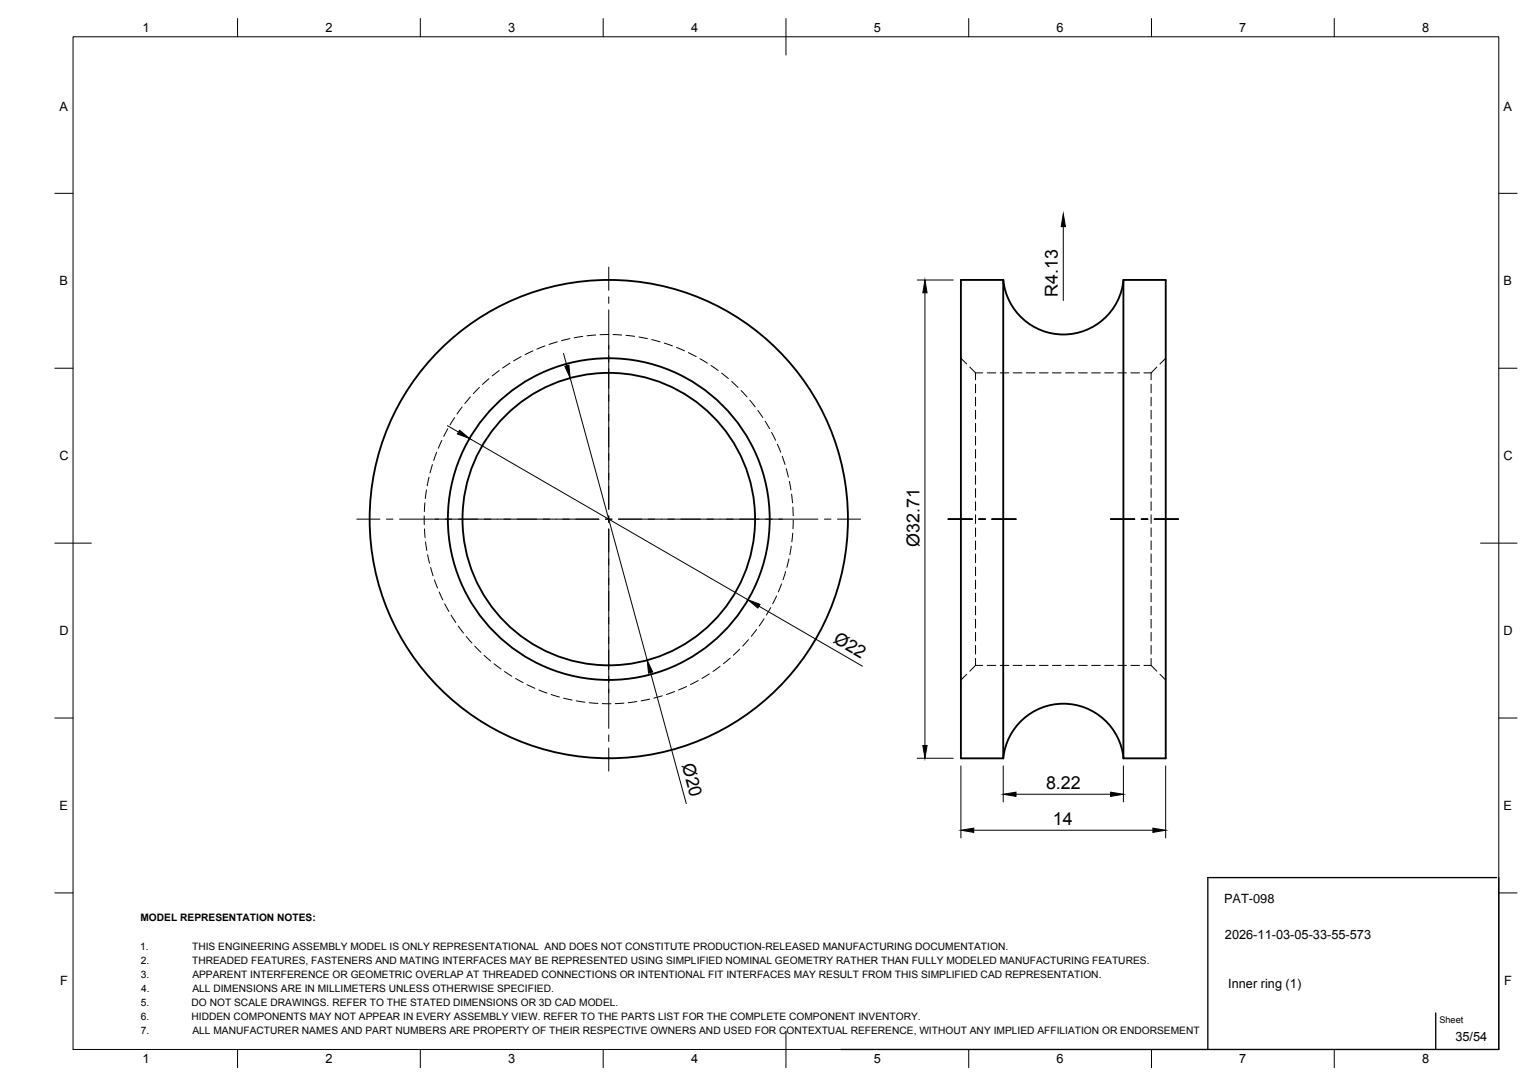
ISO-10303-21;
HEADER;
/* Generated by software containing ST-Developer
 * from STEP Tools, Inc. (www.steptools.com) 
 */

FILE_DESCRIPTION(
/* description */ ('Spring compression tester'),
/* implementation_level */ '2;1');

FILE_NAME(
/* name */ 'Inner ring (1).step',
/* time_stamp */ '2026-10-28T03:24:11-07:00',
/* author */ (''),
/* organization */ (''),
/* preprocessor_version */ 'ST-DEVELOPER v20.2',
/* originating_system */ 'Autodesk Translation Framework v15.17.0.0',
/* authorisation */ '');

FILE_SCHEMA (('AUTOMOTIVE_DESIGN { 1 0 10303 214 3 1 1 }'));
ENDSEC;

DATA;
#10=MECHANICAL_DESIGN_GEOMETRIC_PRESENTATION_REPRESENTATION('',(#1139),#43521);
#929=TOROIDAL_SURFACE('',#20122,1.675,0.412776);
#954=CONICAL_SURFACE('',#20133,1.05,0.785398163397449);
#955=CONICAL_SURFACE('',#20140,1.05,0.785398163397449);
#1012=SHAPE_REPRESENTATION_RELATIONSHIP('SRR','None',#43826,#1072);
#1072=ADVANCED_BREP_SHAPE_REPRESENTATION('',(#1213),#43486);
#1139=STYLED_ITEM('',(#44202),#1213);
#1213=MANIFOLD_SOLID_BREP('Body1',#18577);
#1459=FACE_BOUND('',#3908,.T.);
#1460=FACE_BOUND('',#3911,.T.);
#1904=PLANE('',#20135);
#1905=PLANE('',#20138);
#2644=FACE_OUTER_BOUND('',#3903,.T.);
#2645=FACE_OUTER_BOUND('',#3904,.T.);
#2646=FACE_OUTER_BOUND('',#3905,.T.);
#2647=FACE_OUTER_BOUND('',#3906,.T.);
#2648=FACE_OUTER_BOUND('',#3907,.T.);
#2649=FACE_OUTER_BOUND('',#3909,.T.);
#2650=FACE_OUTER_BOUND('',#3910,.T.);
#2651=FACE_OUTER_BOUND('',#3912,.T.);
#3903=EDGE_LOOP('',(#14319,#14320,#14321,#14322,#14323,#14324));
#3904=EDGE_LOOP('',(#14325,#14326,#14327,#14328,#14329));
#3905=EDGE_LOOP('',(#14330,#14331,#14332,#14333));
#3906=EDGE_LOOP('',(#14334,#14335,#14336,#14337));
#3907=EDGE_LOOP('',(#14338));
#3908=EDGE_LOOP('',(#14339));
#3909=EDGE_LOOP('',(#14340,#14341,#14342,#14343,#14344));
#3910=EDGE_LOOP('',(#14345));
#3911=EDGE_LOOP('',(#14346));
#3912=EDGE_LOOP('',(#14347,#14348,#14349,#14350));
#5317=LINE('',#29028,#6749);
#5318=LINE('',#29034,#6750);
#5319=LINE('',#29038,#6751);
#5320=LINE('',#29044,#6752);
#5321=LINE('',#29049,#6753);
#6749=VECTOR('',#23597,1.63531);
#6750=VECTOR('',#23604,1.);
#6751=VECTOR('',#23609,1.05);
#6752=VECTOR('',#23618,1.63531);
#6753=VECTOR('',#23625,1.05);
#7796=CIRCLE('',#20123,1.63531);
#7797=CIRCLE('',#20124,1.63531);
#7798=CIRCLE('',#20125,0.412776);
#7799=CIRCLE('',#20126,1.63531);
#7800=CIRCLE('',#20127,1.63531);
#7801=CIRCLE('',#20129,1.63531);
#7802=CIRCLE('',#20131,1.);
#7803=CIRCLE('',#20132,1.);
#7804=CIRCLE('',#20134,1.1);
#7805=CIRCLE('',#20137,1.63531);
#7806=CIRCLE('',#20139,1.1);
#8843=VERTEX_POINT('',#29017);
#8844=VERTEX_POINT('',#29018);
#8845=VERTEX_POINT('',#29021);
#8846=VERTEX_POINT('',#29023);
#8847=VERTEX_POINT('',#29027);
#8848=VERTEX_POINT('',#29031);
#8849=VERTEX_POINT('',#29033);
#8850=VERTEX_POINT('',#29037);
#8851=VERTEX_POINT('',#29042);
#8852=VERTEX_POINT('',#29046);
#10824=EDGE_CURVE('',#8843,#8844,#7796,.T.);
#10825=EDGE_CURVE('',#8844,#8843,#7797,.T.);
#10826=EDGE_CURVE('',#8844,#8845,#7798,.T.);
#10827=EDGE_CURVE('',#8846,#8845,#7799,.T.);
#10828=EDGE_CURVE('',#8845,#8846,#7800,.T.);
#10829=EDGE_CURVE('',#8846,#8847,#5317,.T.);
#10830=EDGE_CURVE('',#8847,#8847,#7801,.T.);
#10831=EDGE_CURVE('',#8848,#8848,#7802,.T.);
#10832=EDGE_CURVE('',#8848,#8849,#5318,.T.);
#10833=EDGE_CURVE('',#8849,#8849,#7803,.T.);
#10834=EDGE_CURVE('',#8849,#8850,#5319,.T.);
#10835=EDGE_CURVE('',#8850,#8850,#7804,.T.);
#10836=EDGE_CURVE('',#8851,#8851,#7805,.T.);
#10837=EDGE_CURVE('',#8851,#8843,#5320,.T.);
#10838=EDGE_CURVE('',#8852,#8852,#7806,.T.);
#10839=EDGE_CURVE('',#8852,#8848,#5321,.T.);
#14319=ORIENTED_EDGE('',*,*,#10824,.F.);
#14320=ORIENTED_EDGE('',*,*,#10825,.F.);
#14321=ORIENTED_EDGE('',*,*,#10826,.T.);
#14322=ORIENTED_EDGE('',*,*,#10827,.F.);
#14323=ORIENTED_EDGE('',*,*,#10828,.F.);
#14324=ORIENTED_EDGE('',*,*,#10826,.F.);
#14325=ORIENTED_EDGE('',*,*,#10827,.T.);
#14326=ORIENTED_EDGE('',*,*,#10828,.T.);
#14327=ORIENTED_EDGE('',*,*,#10829,.T.);
#14328=ORIENTED_EDGE('',*,*,#10830,.T.);
#14329=ORIENTED_EDGE('',*,*,#10829,.F.);
#14330=ORIENTED_EDGE('',*,*,#10831,.T.);
#14331=ORIENTED_EDGE('',*,*,#10832,.T.);
#14332=ORIENTED_EDGE('',*,*,#10833,.F.);
#14333=ORIENTED_EDGE('',*,*,#10832,.F.);
#14334=ORIENTED_EDGE('',*,*,#10833,.T.);
#14335=ORIENTED_EDGE('',*,*,#10834,.T.);
#14336=ORIENTED_EDGE('',*,*,#10835,.F.);
#14337=ORIENTED_EDGE('',*,*,#10834,.F.);
#14338=ORIENTED_EDGE('',*,*,#10830,.F.);
#14339=ORIENTED_EDGE('',*,*,#10835,.T.);
#14340=ORIENTED_EDGE('',*,*,#10836,.F.);
#14341=ORIENTED_EDGE('',*,*,#10837,.T.);
#14342=ORIENTED_EDGE('',*,*,#10824,.T.);
#14343=ORIENTED_EDGE('',*,*,#10825,.T.);
#14344=ORIENTED_EDGE('',*,*,#10837,.F.);
#14345=ORIENTED_EDGE('',*,*,#10836,.T.);
#14346=ORIENTED_EDGE('',*,*,#10838,.F.);
#14347=ORIENTED_EDGE('',*,*,#10838,.T.);
#14348=ORIENTED_EDGE('',*,*,#10839,.T.);
#14349=ORIENTED_EDGE('',*,*,#10831,.F.);
#14350=ORIENTED_EDGE('',*,*,#10839,.F.);
#17239=CYLINDRICAL_SURFACE('',#20128,1.63531);
#17240=CYLINDRICAL_SURFACE('',#20130,1.);
#17241=CYLINDRICAL_SURFACE('',#20136,1.63531);
#17968=ADVANCED_FACE('',(#2644),#929,.F.);
#17969=ADVANCED_FACE('',(#2645),#17239,.T.);
#17970=ADVANCED_FACE('',(#2646),#17240,.F.);
#17971=ADVANCED_FACE('',(#2647),#954,.F.);
#17972=ADVANCED_FACE('',(#2648,#1459),#1904,.T.);
#17973=ADVANCED_FACE('',(#2649),#17241,.T.);
#17974=ADVANCED_FACE('',(#2650,#1460),#1905,.T.);
#17975=ADVANCED_FACE('',(#2651),#955,.F.);
#18577=CLOSED_SHELL('',(#17968,#17969,#17970,#17971,#17972,#17973,#17974,
#17975));
#20121=AXIS2_PLACEMENT_3D('',#29015,#23581,#23582);
#20122=AXIS2_PLACEMENT_3D('',#29016,#23583,#23584);
#20123=AXIS2_PLACEMENT_3D('',#29019,#23585,#23586);
#20124=AXIS2_PLACEMENT_3D('',#29020,#23587,#23588);
#20125=AXIS2_PLACEMENT_3D('',#29022,#23589,#23590);
#20126=AXIS2_PLACEMENT_3D('',#29024,#23591,#23592);
#20127=AXIS2_PLACEMENT_3D('',#29025,#23593,#23594);
#20128=AXIS2_PLACEMENT_3D('',#29026,#23595,#23596);
#20129=AXIS2_PLACEMENT_3D('',#29029,#23598,#23599);
#20130=AXIS2_PLACEMENT_3D('',#29030,#23600,#23601);
#20131=AXIS2_PLACEMENT_3D('',#29032,#23602,#23603);
#20132=AXIS2_PLACEMENT_3D('',#29035,#23605,#23606);
#20133=AXIS2_PLACEMENT_3D('',#29036,#23607,#23608);
#20134=AXIS2_PLACEMENT_3D('',#29039,#23610,#23611);
#20135=AXIS2_PLACEMENT_3D('',#29040,#23612,#23613);
#20136=AXIS2_PLACEMENT_3D('',#29041,#23614,#23615);
#20137=AXIS2_PLACEMENT_3D('',#29043,#23616,#23617);
#20138=AXIS2_PLACEMENT_3D('',#29045,#23619,#23620);
#20139=AXIS2_PLACEMENT_3D('',#29047,#23621,#23622);
#20140=AXIS2_PLACEMENT_3D('',#29048,#23623,#23624);
#23581=DIRECTION('axis',(0.,0.,1.));
#23582=DIRECTION('refdir',(1.,0.,0.));
#23583=DIRECTION('center_axis',(0.,-1.,0.));
#23584=DIRECTION('ref_axis',(0.,0.,-1.));
#23585=DIRECTION('center_axis',(0.,-1.,0.));
#23586=DIRECTION('ref_axis',(1.,0.,0.));
#23587=DIRECTION('center_axis',(0.,-1.,0.));
#23588=DIRECTION('ref_axis',(1.,0.,0.));
#23589=DIRECTION('center_axis',(1.,0.,1.22464679914735E-16));
#23590=DIRECTION('ref_axis',(-1.22464679914735E-16,0.,1.));
#23591=DIRECTION('center_axis',(0.,1.,0.));
#23592=DIRECTION('ref_axis',(1.,0.,0.));
#23593=DIRECTION('center_axis',(0.,1.,0.));
#23594=DIRECTION('ref_axis',(1.,0.,0.));
#23595=DIRECTION('center_axis',(0.,-1.,0.));
#23596=DIRECTION('ref_axis',(1.,0.,0.));
#23597=DIRECTION('',(0.,1.,0.));
#23598=DIRECTION('center_axis',(0.,-1.,0.));
#23599=DIRECTION('ref_axis',(1.,0.,0.));
#23600=DIRECTION('center_axis',(0.,-1.,0.));
#23601=DIRECTION('ref_axis',(1.,0.,0.));
#23602=DIRECTION('center_axis',(0.,-1.,0.));
#23603=DIRECTION('ref_axis',(1.,0.,0.));
#23604=DIRECTION('',(0.,1.,0.));
#23605=DIRECTION('center_axis',(0.,-1.,0.));
#23606=DIRECTION('ref_axis',(1.,0.,0.));
#23607=DIRECTION('center_axis',(0.,1.,0.));
#23608=DIRECTION('ref_axis',(1.,0.,0.));
#23609=DIRECTION('',(-0.707106781186548,0.707106781186547,-8.65956056235494E-17));
#23610=DIRECTION('center_axis',(0.,-1.,0.));
#23611=DIRECTION('ref_axis',(1.,0.,0.));
#23612=DIRECTION('center_axis',(0.,1.,0.));
#23613=DIRECTION('ref_axis',(0.,0.,1.));
#23614=DIRECTION('center_axis',(0.,-1.,0.));
#23615=DIRECTION('ref_axis',(1.,0.,0.));
#23616=DIRECTION('center_axis',(0.,-1.,0.));
#23617=DIRECTION('ref_axis',(1.,0.,0.));
#23618=DIRECTION('',(0.,1.,0.));
#23619=DIRECTION('center_axis',(0.,-1.,0.));
#23620=DIRECTION('ref_axis',(0.,0.,-1.));
#23621=DIRECTION('center_axis',(0.,-1.,0.));
#23622=DIRECTION('ref_axis',(1.,0.,0.));
#23623=DIRECTION('center_axis',(0.,-1.,0.));
#23624=DIRECTION('ref_axis',(1.,0.,0.));
#23625=DIRECTION('',(0.707106781186548,0.707106781186547,8.65956056235494E-17));
#29015=CARTESIAN_POINT('',(0.,0.,0.));
#29016=CARTESIAN_POINT('Origin',(0.,0.,0.));
#29017=CARTESIAN_POINT('',(-1.63531,-0.410863395882378,-2.00267715711366E-16));
#29018=CARTESIAN_POINT('',(-2.00267715711366E-16,-0.410863395882378,1.63531));
#29019=CARTESIAN_POINT('Origin',(0.,-0.410863395882378,0.));
#29020=CARTESIAN_POINT('Origin',(0.,-0.410863395882378,0.));
#29021=CARTESIAN_POINT('',(-2.00267715711366E-16,0.410863395882378,1.63531));
#29022=CARTESIAN_POINT('Origin',(-2.05128338857182E-16,0.,1.675));
#29023=CARTESIAN_POINT('',(-1.63531,0.410863395882378,2.00267715711366E-16));
#29024=CARTESIAN_POINT('Origin',(0.,0.410863395882378,0.));
#29025=CARTESIAN_POINT('Origin',(0.,0.410863395882378,0.));
#29026=CARTESIAN_POINT('Origin',(0.,0.,0.));
#29027=CARTESIAN_POINT('',(-1.63531,0.7,-2.00267715711366E-16));
#29028=CARTESIAN_POINT('',(-1.63531,0.,-2.00267715711366E-16));
#29029=CARTESIAN_POINT('Origin',(0.,0.7,0.));
#29030=CARTESIAN_POINT('Origin',(0.,0.,0.));
#29031=CARTESIAN_POINT('',(-1.,-0.6,-1.22464679914735E-16));
#29032=CARTESIAN_POINT('Origin',(0.,-0.6,0.));
#29033=CARTESIAN_POINT('',(-1.,0.6,-1.22464679914735E-16));
#29034=CARTESIAN_POINT('',(-1.,0.,-1.22464679914735E-16));
#29035=CARTESIAN_POINT('Origin',(0.,0.6,0.));
#29036=CARTESIAN_POINT('Origin',(0.,0.65,0.));
#29037=CARTESIAN_POINT('',(-1.1,0.7,-1.34711147906209E-16));
#29038=CARTESIAN_POINT('',(-1.05,0.65,-1.28587913910472E-16));
#29039=CARTESIAN_POINT('Origin',(0.,0.7,0.));
#29040=CARTESIAN_POINT('Origin',(1.63531,0.7,0.));
#29041=CARTESIAN_POINT('Origin',(0.,0.,0.));
#29042=CARTESIAN_POINT('',(-1.63531,-0.7,-2.00267715711366E-16));
#29043=CARTESIAN_POINT('Origin',(0.,-0.7,0.));
#29044=CARTESIAN_POINT('',(-1.63531,0.,-2.00267715711366E-16));
#29045=CARTESIAN_POINT('Origin',(1.1,-0.7,0.));
#29046=CARTESIAN_POINT('',(-1.1,-0.7,-1.34711147906209E-16));
#29047=CARTESIAN_POINT('Origin',(0.,-0.7,0.));
#29048=CARTESIAN_POINT('Origin',(0.,-0.65,0.));
#29049=CARTESIAN_POINT('',(-1.05,-0.65,-1.28587913910472E-16));
#43418=UNCERTAINTY_MEASURE_WITH_UNIT(LENGTH_MEASURE(0.001),#43522,
'DISTANCE_ACCURACY_VALUE',
'Maximum model space distance between geometric entities at asserted c
onnectivities');
#43453=UNCERTAINTY_MEASURE_WITH_UNIT(LENGTH_MEASURE(0.001),#43522,
'DISTANCE_ACCURACY_VALUE',
'Maximum model space distance between geometric entities at asserted c
onnectivities');
#43486=(
GEOMETRIC_REPRESENTATION_CONTEXT(3)
GLOBAL_UNCERTAINTY_ASSIGNED_CONTEXT((#43418))
GLOBAL_UNIT_ASSIGNED_CONTEXT((#43522,#43524,#43525))
REPRESENTATION_CONTEXT('','3D')
);
#43521=(
GEOMETRIC_REPRESENTATION_CONTEXT(3)
GLOBAL_UNCERTAINTY_ASSIGNED_CONTEXT((#43453))
GLOBAL_UNIT_ASSIGNED_CONTEXT((#43522,#43524,#43525))
REPRESENTATION_CONTEXT('','3D')
);
#43522=(
LENGTH_UNIT()
NAMED_UNIT(*)
SI_UNIT(.CENTI.,.METRE.)
);
#43524=(
NAMED_UNIT(*)
PLANE_ANGLE_UNIT()
SI_UNIT($,.RADIAN.)
);
#43525=(
NAMED_UNIT(*)
SI_UNIT($,.STERADIAN.)
SOLID_ANGLE_UNIT()
);
#43558=SHAPE_DEFINITION_REPRESENTATION(#43630,#43826);
#43630=PRODUCT_DEFINITION_SHAPE('',$,#43894);
#43826=SHAPE_REPRESENTATION('',(#20121),#43486);
#43861=PRODUCT_DEFINITION_CONTEXT('part definition',#44064,'design');
#43894=PRODUCT_DEFINITION('Inner ring (1)','Inner ring (1)',#43961,#43861);
#43961=PRODUCT_DEFINITION_FORMATION('',$,#44098);
#44064=APPLICATION_CONTEXT(
'Core Data for Automotive Mechanical Design Process');
#44065=PRODUCT_CONTEXT('part definition',#44064,'mechanical');
#44098=PRODUCT('Inner ring (1)','Inner ring (1)','Inner ring (1)',(#44065));
#44196=COLOUR_RGB('Grey',0.48,0.52,0.57);
#44197=FILL_AREA_STYLE_COLOUR('',#44196);
#44198=FILL_AREA_STYLE('',(#44197));
#44199=SURFACE_STYLE_FILL_AREA(#44198);
#44200=SURFACE_SIDE_STYLE('',(#44199));
#44201=SURFACE_STYLE_USAGE(.BOTH.,#44200);
#44202=PRESENTATION_STYLE_ASSIGNMENT((#44201));
ENDSEC;
END-ISO-10303-21;
